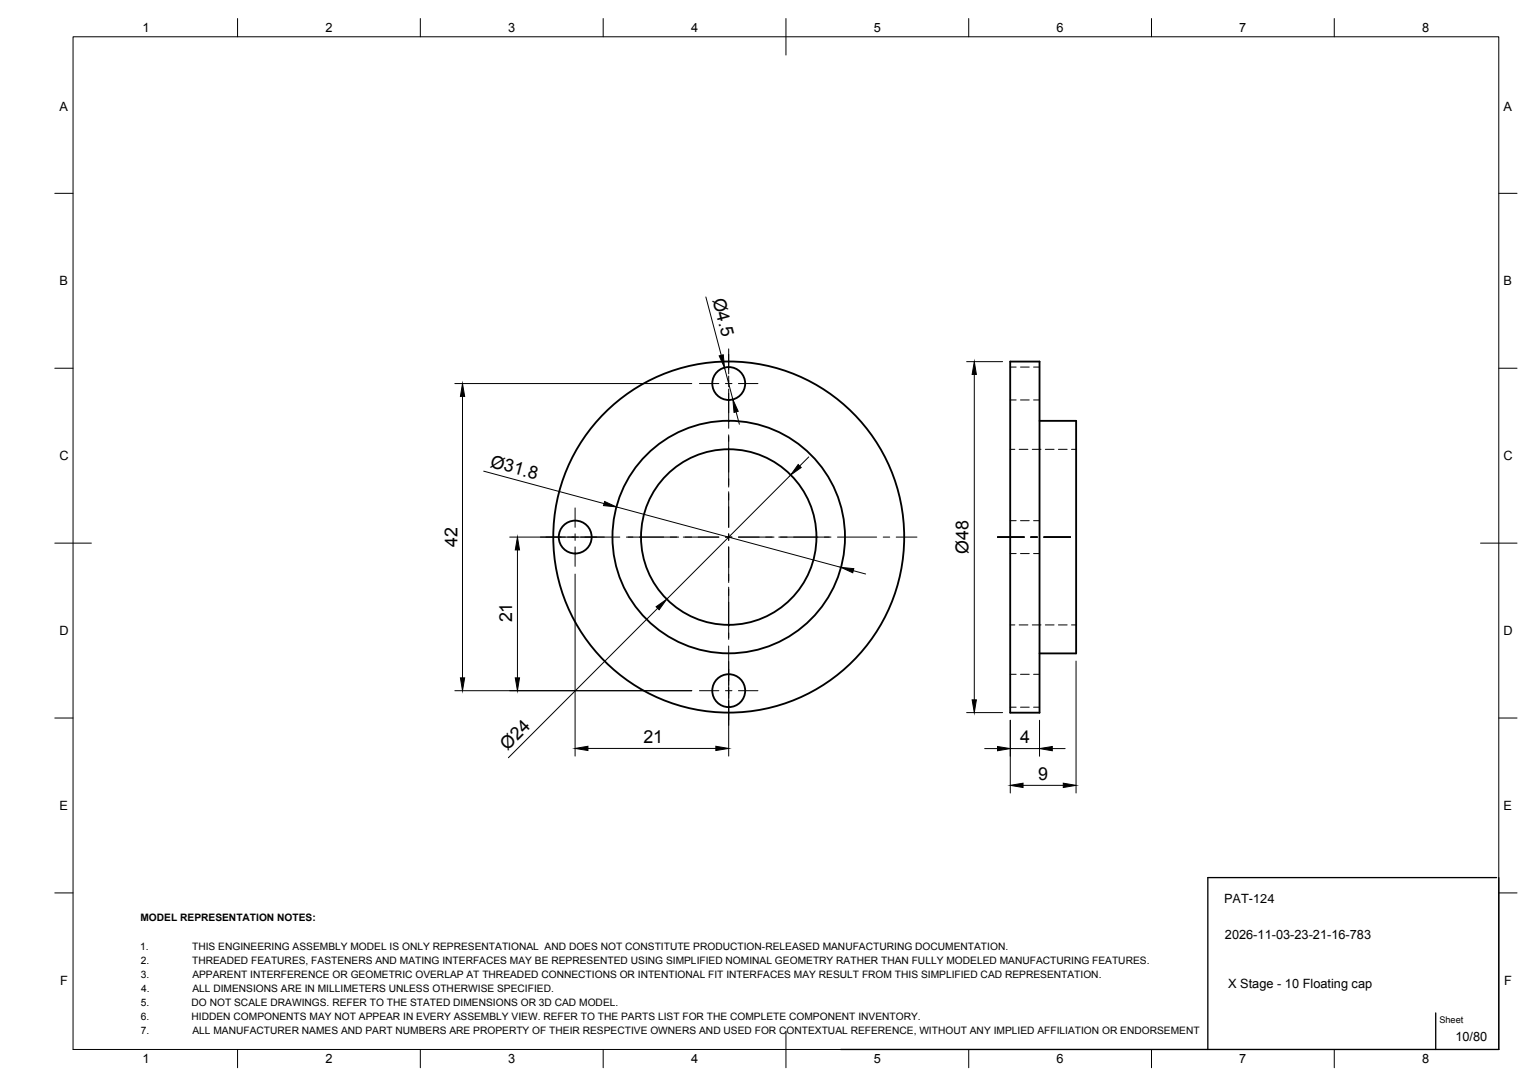
ISO-10303-21;
HEADER;
/* Generated by software containing ST-Developer
 * from STEP Tools, Inc. (www.steptools.com) 
 */

FILE_DESCRIPTION(
/* description */ ('XY cross-slide table'),
/* implementation_level */ '2;1');

FILE_NAME(
/* name */ 'X Stage - 10 Floating cap.step',
/* time_stamp */ '2026-10-28T03:22:46-07:00',
/* author */ (''),
/* organization */ (''),
/* preprocessor_version */ 'ST-DEVELOPER v20.2',
/* originating_system */ 'Autodesk Translation Framework v15.17.0.0',
/* authorisation */ '');

FILE_SCHEMA (('AUTOMOTIVE_DESIGN { 1 0 10303 214 3 1 1 }'));
ENDSEC;

DATA;
#10=MECHANICAL_DESIGN_GEOMETRIC_PRESENTATION_REPRESENTATION('',(#1675),#62984);
#1509=SHAPE_REPRESENTATION_RELATIONSHIP('SRR','None',#63357,#1592);
#1592=ADVANCED_BREP_SHAPE_REPRESENTATION('',(#1788),#62894);
#1675=STYLED_ITEM('',(#63926),#1788);
#1788=MANIFOLD_SOLID_BREP('Body1',#22969);
#1936=FACE_BOUND('',#4305,.T.);
#1937=FACE_BOUND('',#4309,.T.);
#1938=FACE_BOUND('',#4310,.T.);
#1939=FACE_BOUND('',#4311,.T.);
#1940=FACE_BOUND('',#4312,.T.);
#1941=FACE_BOUND('',#4314,.T.);
#1942=FACE_BOUND('',#4315,.T.);
#1943=FACE_BOUND('',#4316,.T.);
#1944=FACE_BOUND('',#4317,.T.);
#2333=PLANE('',#24151);
#2334=PLANE('',#24158);
#2335=PLANE('',#24159);
#2937=FACE_OUTER_BOUND('',#4300,.T.);
#2938=FACE_OUTER_BOUND('',#4301,.T.);
#2939=FACE_OUTER_BOUND('',#4302,.T.);
#2940=FACE_OUTER_BOUND('',#4303,.T.);
#2941=FACE_OUTER_BOUND('',#4304,.T.);
#2942=FACE_OUTER_BOUND('',#4306,.T.);
#2943=FACE_OUTER_BOUND('',#4307,.T.);
#2944=FACE_OUTER_BOUND('',#4308,.T.);
#2945=FACE_OUTER_BOUND('',#4313,.T.);
#4300=EDGE_LOOP('',(#15218,#15219,#15220,#15221));
#4301=EDGE_LOOP('',(#15222,#15223,#15224,#15225));
#4302=EDGE_LOOP('',(#15226,#15227,#15228,#15229));
#4303=EDGE_LOOP('',(#15230,#15231,#15232,#15233));
#4304=EDGE_LOOP('',(#15234));
#4305=EDGE_LOOP('',(#15235));
#4306=EDGE_LOOP('',(#15236,#15237,#15238,#15239));
#4307=EDGE_LOOP('',(#15240,#15241,#15242,#15243));
#4308=EDGE_LOOP('',(#15244));
#4309=EDGE_LOOP('',(#15245));
#4310=EDGE_LOOP('',(#15246));
#4311=EDGE_LOOP('',(#15247));
#4312=EDGE_LOOP('',(#15248));
#4313=EDGE_LOOP('',(#15249));
#4314=EDGE_LOOP('',(#15250));
#4315=EDGE_LOOP('',(#15251));
#4316=EDGE_LOOP('',(#15252));
#4317=EDGE_LOOP('',(#15253));
#6001=LINE('',#33210,#7488);
#6002=LINE('',#33216,#7489);
#6003=LINE('',#33222,#7490);
#6004=LINE('',#33228,#7491);
#6005=LINE('',#33235,#7492);
#6006=LINE('',#33241,#7493);
#7488=VECTOR('',#26838,0.225);
#7489=VECTOR('',#26845,0.225);
#7490=VECTOR('',#26852,0.225);
#7491=VECTOR('',#26859,1.59);
#7492=VECTOR('',#26868,1.2);
#7493=VECTOR('',#26875,2.4);
#8942=CIRCLE('',#24140,0.225);
#8943=CIRCLE('',#24141,0.225);
#8944=CIRCLE('',#24143,0.225);
#8945=CIRCLE('',#24144,0.225);
#8946=CIRCLE('',#24146,0.225);
#8947=CIRCLE('',#24147,0.225);
#8948=CIRCLE('',#24149,1.59);
#8949=CIRCLE('',#24150,1.59);
#8950=CIRCLE('',#24152,1.2);
#8951=CIRCLE('',#24154,1.2);
#8952=CIRCLE('',#24156,2.4);
#8953=CIRCLE('',#24157,2.4);
#9875=VERTEX_POINT('',#33207);
#9876=VERTEX_POINT('',#33209);
#9877=VERTEX_POINT('',#33213);
#9878=VERTEX_POINT('',#33215);
#9879=VERTEX_POINT('',#33219);
#9880=VERTEX_POINT('',#33221);
#9881=VERTEX_POINT('',#33225);
#9882=VERTEX_POINT('',#33227);
#9883=VERTEX_POINT('',#33231);
#9884=VERTEX_POINT('',#33234);
#9885=VERTEX_POINT('',#33238);
#9886=VERTEX_POINT('',#33240);
#11993=EDGE_CURVE('',#9875,#9875,#8942,.T.);
#11994=EDGE_CURVE('',#9875,#9876,#6001,.T.);
#11995=EDGE_CURVE('',#9876,#9876,#8943,.T.);
#11996=EDGE_CURVE('',#9877,#9877,#8944,.T.);
#11997=EDGE_CURVE('',#9877,#9878,#6002,.T.);
#11998=EDGE_CURVE('',#9878,#9878,#8945,.T.);
#11999=EDGE_CURVE('',#9879,#9879,#8946,.T.);
#12000=EDGE_CURVE('',#9879,#9880,#6003,.T.);
#12001=EDGE_CURVE('',#9880,#9880,#8947,.T.);
#12002=EDGE_CURVE('',#9881,#9881,#8948,.T.);
#12003=EDGE_CURVE('',#9881,#9882,#6004,.T.);
#12004=EDGE_CURVE('',#9882,#9882,#8949,.T.);
#12005=EDGE_CURVE('',#9883,#9883,#8950,.T.);
#12006=EDGE_CURVE('',#9883,#9884,#6005,.T.);
#12007=EDGE_CURVE('',#9884,#9884,#8951,.T.);
#12008=EDGE_CURVE('',#9885,#9885,#8952,.T.);
#12009=EDGE_CURVE('',#9885,#9886,#6006,.T.);
#12010=EDGE_CURVE('',#9886,#9886,#8953,.T.);
#15218=ORIENTED_EDGE('',*,*,#11993,.F.);
#15219=ORIENTED_EDGE('',*,*,#11994,.T.);
#15220=ORIENTED_EDGE('',*,*,#11995,.F.);
#15221=ORIENTED_EDGE('',*,*,#11994,.F.);
#15222=ORIENTED_EDGE('',*,*,#11996,.F.);
#15223=ORIENTED_EDGE('',*,*,#11997,.T.);
#15224=ORIENTED_EDGE('',*,*,#11998,.F.);
#15225=ORIENTED_EDGE('',*,*,#11997,.F.);
#15226=ORIENTED_EDGE('',*,*,#11999,.F.);
#15227=ORIENTED_EDGE('',*,*,#12000,.T.);
#15228=ORIENTED_EDGE('',*,*,#12001,.F.);
#15229=ORIENTED_EDGE('',*,*,#12000,.F.);
#15230=ORIENTED_EDGE('',*,*,#12002,.F.);
#15231=ORIENTED_EDGE('',*,*,#12003,.T.);
#15232=ORIENTED_EDGE('',*,*,#12004,.F.);
#15233=ORIENTED_EDGE('',*,*,#12003,.F.);
#15234=ORIENTED_EDGE('',*,*,#12002,.T.);
#15235=ORIENTED_EDGE('',*,*,#12005,.T.);
#15236=ORIENTED_EDGE('',*,*,#12005,.F.);
#15237=ORIENTED_EDGE('',*,*,#12006,.T.);
#15238=ORIENTED_EDGE('',*,*,#12007,.T.);
#15239=ORIENTED_EDGE('',*,*,#12006,.F.);
#15240=ORIENTED_EDGE('',*,*,#12008,.F.);
#15241=ORIENTED_EDGE('',*,*,#12009,.T.);
#15242=ORIENTED_EDGE('',*,*,#12010,.T.);
#15243=ORIENTED_EDGE('',*,*,#12009,.F.);
#15244=ORIENTED_EDGE('',*,*,#12008,.T.);
#15245=ORIENTED_EDGE('',*,*,#11995,.T.);
#15246=ORIENTED_EDGE('',*,*,#11998,.T.);
#15247=ORIENTED_EDGE('',*,*,#12001,.T.);
#15248=ORIENTED_EDGE('',*,*,#12004,.T.);
#15249=ORIENTED_EDGE('',*,*,#12010,.F.);
#15250=ORIENTED_EDGE('',*,*,#11993,.T.);
#15251=ORIENTED_EDGE('',*,*,#11996,.T.);
#15252=ORIENTED_EDGE('',*,*,#11999,.T.);
#15253=ORIENTED_EDGE('',*,*,#12007,.F.);
#21071=CYLINDRICAL_SURFACE('',#24139,0.225);
#21072=CYLINDRICAL_SURFACE('',#24142,0.225);
#21073=CYLINDRICAL_SURFACE('',#24145,0.225);
#21074=CYLINDRICAL_SURFACE('',#24148,1.59);
#21075=CYLINDRICAL_SURFACE('',#24153,1.2);
#21076=CYLINDRICAL_SURFACE('',#24155,2.4);
#21718=ADVANCED_FACE('',(#2937),#21071,.F.);
#21719=ADVANCED_FACE('',(#2938),#21072,.F.);
#21720=ADVANCED_FACE('',(#2939),#21073,.F.);
#21721=ADVANCED_FACE('',(#2940),#21074,.T.);
#21722=ADVANCED_FACE('',(#2941,#1936),#2333,.T.);
#21723=ADVANCED_FACE('',(#2942),#21075,.F.);
#21724=ADVANCED_FACE('',(#2943),#21076,.T.);
#21725=ADVANCED_FACE('',(#2944,#1937,#1938,#1939,#1940),#2334,.T.);
#21726=ADVANCED_FACE('',(#2945,#1941,#1942,#1943,#1944),#2335,.F.);
#22969=CLOSED_SHELL('',(#21718,#21719,#21720,#21721,#21722,#21723,#21724,
#21725,#21726));
#24138=AXIS2_PLACEMENT_3D('',#33205,#26832,#26833);
#24139=AXIS2_PLACEMENT_3D('',#33206,#26834,#26835);
#24140=AXIS2_PLACEMENT_3D('',#33208,#26836,#26837);
#24141=AXIS2_PLACEMENT_3D('',#33211,#26839,#26840);
#24142=AXIS2_PLACEMENT_3D('',#33212,#26841,#26842);
#24143=AXIS2_PLACEMENT_3D('',#33214,#26843,#26844);
#24144=AXIS2_PLACEMENT_3D('',#33217,#26846,#26847);
#24145=AXIS2_PLACEMENT_3D('',#33218,#26848,#26849);
#24146=AXIS2_PLACEMENT_3D('',#33220,#26850,#26851);
#24147=AXIS2_PLACEMENT_3D('',#33223,#26853,#26854);
#24148=AXIS2_PLACEMENT_3D('',#33224,#26855,#26856);
#24149=AXIS2_PLACEMENT_3D('',#33226,#26857,#26858);
#24150=AXIS2_PLACEMENT_3D('',#33229,#26860,#26861);
#24151=AXIS2_PLACEMENT_3D('',#33230,#26862,#26863);
#24152=AXIS2_PLACEMENT_3D('',#33232,#26864,#26865);
#24153=AXIS2_PLACEMENT_3D('',#33233,#26866,#26867);
#24154=AXIS2_PLACEMENT_3D('',#33236,#26869,#26870);
#24155=AXIS2_PLACEMENT_3D('',#33237,#26871,#26872);
#24156=AXIS2_PLACEMENT_3D('',#33239,#26873,#26874);
#24157=AXIS2_PLACEMENT_3D('',#33242,#26876,#26877);
#24158=AXIS2_PLACEMENT_3D('',#33243,#26878,#26879);
#24159=AXIS2_PLACEMENT_3D('',#33244,#26880,#26881);
#26832=DIRECTION('axis',(0.,0.,1.));
#26833=DIRECTION('refdir',(1.,0.,0.));
#26834=DIRECTION('center_axis',(1.,0.,0.));
#26835=DIRECTION('ref_axis',(0.,0.,-1.));
#26836=DIRECTION('center_axis',(1.,0.,0.));
#26837=DIRECTION('ref_axis',(0.,0.,-1.));
#26838=DIRECTION('',(1.,0.,0.));
#26839=DIRECTION('center_axis',(-1.,0.,0.));
#26840=DIRECTION('ref_axis',(0.,0.,-1.));
#26841=DIRECTION('center_axis',(1.,0.,0.));
#26842=DIRECTION('ref_axis',(0.,0.,-1.));
#26843=DIRECTION('center_axis',(1.,0.,0.));
#26844=DIRECTION('ref_axis',(0.,0.,-1.));
#26845=DIRECTION('',(1.,0.,0.));
#26846=DIRECTION('center_axis',(-1.,0.,0.));
#26847=DIRECTION('ref_axis',(0.,0.,-1.));
#26848=DIRECTION('center_axis',(1.,0.,0.));
#26849=DIRECTION('ref_axis',(0.,0.,-1.));
#26850=DIRECTION('center_axis',(1.,0.,0.));
#26851=DIRECTION('ref_axis',(0.,0.,-1.));
#26852=DIRECTION('',(1.,0.,0.));
#26853=DIRECTION('center_axis',(-1.,0.,0.));
#26854=DIRECTION('ref_axis',(0.,0.,-1.));
#26855=DIRECTION('center_axis',(1.,0.,0.));
#26856=DIRECTION('ref_axis',(0.,0.,-1.));
#26857=DIRECTION('center_axis',(1.,0.,0.));
#26858=DIRECTION('ref_axis',(0.,0.,-1.));
#26859=DIRECTION('',(-1.,0.,0.));
#26860=DIRECTION('center_axis',(-1.,0.,0.));
#26861=DIRECTION('ref_axis',(0.,0.,-1.));
#26862=DIRECTION('center_axis',(1.,0.,0.));
#26863=DIRECTION('ref_axis',(0.,0.,-1.));
#26864=DIRECTION('center_axis',(-1.,0.,0.));
#26865=DIRECTION('ref_axis',(0.,0.,-1.));
#26866=DIRECTION('center_axis',(1.,0.,0.));
#26867=DIRECTION('ref_axis',(0.,0.,-1.));
#26868=DIRECTION('',(-1.,0.,0.));
#26869=DIRECTION('center_axis',(-1.,0.,0.));
#26870=DIRECTION('ref_axis',(0.,0.,-1.));
#26871=DIRECTION('center_axis',(1.,0.,0.));
#26872=DIRECTION('ref_axis',(0.,0.,-1.));
#26873=DIRECTION('center_axis',(1.,0.,0.));
#26874=DIRECTION('ref_axis',(0.,0.,-1.));
#26875=DIRECTION('',(-1.,0.,0.));
#26876=DIRECTION('center_axis',(1.,0.,0.));
#26877=DIRECTION('ref_axis',(0.,0.,-1.));
#26878=DIRECTION('center_axis',(1.,0.,0.));
#26879=DIRECTION('ref_axis',(0.,0.,-1.));
#26880=DIRECTION('center_axis',(1.,0.,0.));
#26881=DIRECTION('ref_axis',(0.,0.,-1.));
#33205=CARTESIAN_POINT('',(0.,0.,0.));
#33206=CARTESIAN_POINT('Origin',(1.5,-2.1,4.));
#33207=CARTESIAN_POINT('',(1.6,-2.1,4.225));
#33208=CARTESIAN_POINT('Origin',(1.6,-2.1,4.));
#33209=CARTESIAN_POINT('',(2.,-2.1,4.225));
#33210=CARTESIAN_POINT('',(1.5,-2.1,4.225));
#33211=CARTESIAN_POINT('Origin',(2.,-2.1,4.));
#33212=CARTESIAN_POINT('Origin',(1.5,2.1,4.));
#33213=CARTESIAN_POINT('',(1.6,2.1,4.225));
#33214=CARTESIAN_POINT('Origin',(1.6,2.1,4.));
#33215=CARTESIAN_POINT('',(2.,2.1,4.225));
#33216=CARTESIAN_POINT('',(1.5,2.1,4.225));
#33217=CARTESIAN_POINT('Origin',(2.,2.1,4.));
#33218=CARTESIAN_POINT('Origin',(1.5,0.,6.1));
#33219=CARTESIAN_POINT('',(1.6,-2.75545529808154E-17,6.325));
#33220=CARTESIAN_POINT('Origin',(1.6,0.,6.1));
#33221=CARTESIAN_POINT('',(2.,2.75545529808154E-17,6.325));
#33222=CARTESIAN_POINT('',(1.5,-2.75545529808154E-17,6.325));
#33223=CARTESIAN_POINT('Origin',(2.,0.,6.1));
#33224=CARTESIAN_POINT('Origin',(2.,0.,4.));
#33225=CARTESIAN_POINT('',(2.5,-1.94718841064429E-16,5.59));
#33226=CARTESIAN_POINT('Origin',(2.5,0.,4.));
#33227=CARTESIAN_POINT('',(2.,-1.94718841064429E-16,5.59));
#33228=CARTESIAN_POINT('',(2.,-1.94718841064429E-16,5.59));
#33229=CARTESIAN_POINT('Origin',(2.,0.,4.));
#33230=CARTESIAN_POINT('Origin',(2.5,0.,4.));
#33231=CARTESIAN_POINT('',(2.5,-1.46957615897682E-16,5.2));
#33232=CARTESIAN_POINT('Origin',(2.5,0.,4.));
#33233=CARTESIAN_POINT('Origin',(1.6,0.,4.));
#33234=CARTESIAN_POINT('',(1.6,-1.46957615897682E-16,5.2));
#33235=CARTESIAN_POINT('',(1.6,-1.46957615897682E-16,5.2));
#33236=CARTESIAN_POINT('Origin',(1.6,0.,4.));
#33237=CARTESIAN_POINT('Origin',(1.6,0.,4.));
#33238=CARTESIAN_POINT('',(2.,-2.93915231795365E-16,6.4));
#33239=CARTESIAN_POINT('Origin',(2.,0.,4.));
#33240=CARTESIAN_POINT('',(1.6,-2.93915231795365E-16,6.4));
#33241=CARTESIAN_POINT('',(1.6,-2.93915231795365E-16,6.4));
#33242=CARTESIAN_POINT('Origin',(1.6,0.,4.));
#33243=CARTESIAN_POINT('Origin',(2.,0.,4.));
#33244=CARTESIAN_POINT('Origin',(1.6,0.,4.));
#62795=UNCERTAINTY_MEASURE_WITH_UNIT(LENGTH_MEASURE(0.001),#62985,
'DISTANCE_ACCURACY_VALUE',
'Maximum model space distance between geometric entities at asserted c
onnectivities');
#62885=UNCERTAINTY_MEASURE_WITH_UNIT(LENGTH_MEASURE(0.001),#62985,
'DISTANCE_ACCURACY_VALUE',
'Maximum model space distance between geometric entities at asserted c
onnectivities');
#62894=(
GEOMETRIC_REPRESENTATION_CONTEXT(3)
GLOBAL_UNCERTAINTY_ASSIGNED_CONTEXT((#62795))
GLOBAL_UNIT_ASSIGNED_CONTEXT((#62985,#62987,#62988))
REPRESENTATION_CONTEXT('','3D')
);
#62984=(
GEOMETRIC_REPRESENTATION_CONTEXT(3)
GLOBAL_UNCERTAINTY_ASSIGNED_CONTEXT((#62885))
GLOBAL_UNIT_ASSIGNED_CONTEXT((#62985,#62987,#62988))
REPRESENTATION_CONTEXT('','3D')
);
#62985=(
LENGTH_UNIT()
NAMED_UNIT(*)
SI_UNIT(.CENTI.,.METRE.)
);
#62987=(
NAMED_UNIT(*)
PLANE_ANGLE_UNIT()
SI_UNIT($,.RADIAN.)
);
#62988=(
NAMED_UNIT(*)
SI_UNIT($,.STERADIAN.)
SOLID_ANGLE_UNIT()
);
#62997=SHAPE_DEFINITION_REPRESENTATION(#63095,#63357);
#63095=PRODUCT_DEFINITION_SHAPE('',$,#63456);
#63357=SHAPE_REPRESENTATION('',(#24138),#62894);
#63447=PRODUCT_DEFINITION_CONTEXT('part definition',#63743,'design');
#63456=PRODUCT_DEFINITION('X Stage - 10 Floating cap',
'X Stage - 10 Floating cap',#63554,#63447);
#63554=PRODUCT_DEFINITION_FORMATION('',$,#63753);
#63743=APPLICATION_CONTEXT(
'Core Data for Automotive Mechanical Design Process');
#63744=PRODUCT_CONTEXT('part definition',#63743,'mechanical');
#63753=PRODUCT('X Stage - 10 Floating cap','X Stage - 10 Floating cap',
'X Stage - 10 Floating cap',(#63744));
#63920=COLOUR_RGB('Off White',0.89,0.88,0.83);
#63921=FILL_AREA_STYLE_COLOUR('',#63920);
#63922=FILL_AREA_STYLE('',(#63921));
#63923=SURFACE_STYLE_FILL_AREA(#63922);
#63924=SURFACE_SIDE_STYLE('',(#63923));
#63925=SURFACE_STYLE_USAGE(.BOTH.,#63924);
#63926=PRESENTATION_STYLE_ASSIGNMENT((#63925));
ENDSEC;
END-ISO-10303-21;
